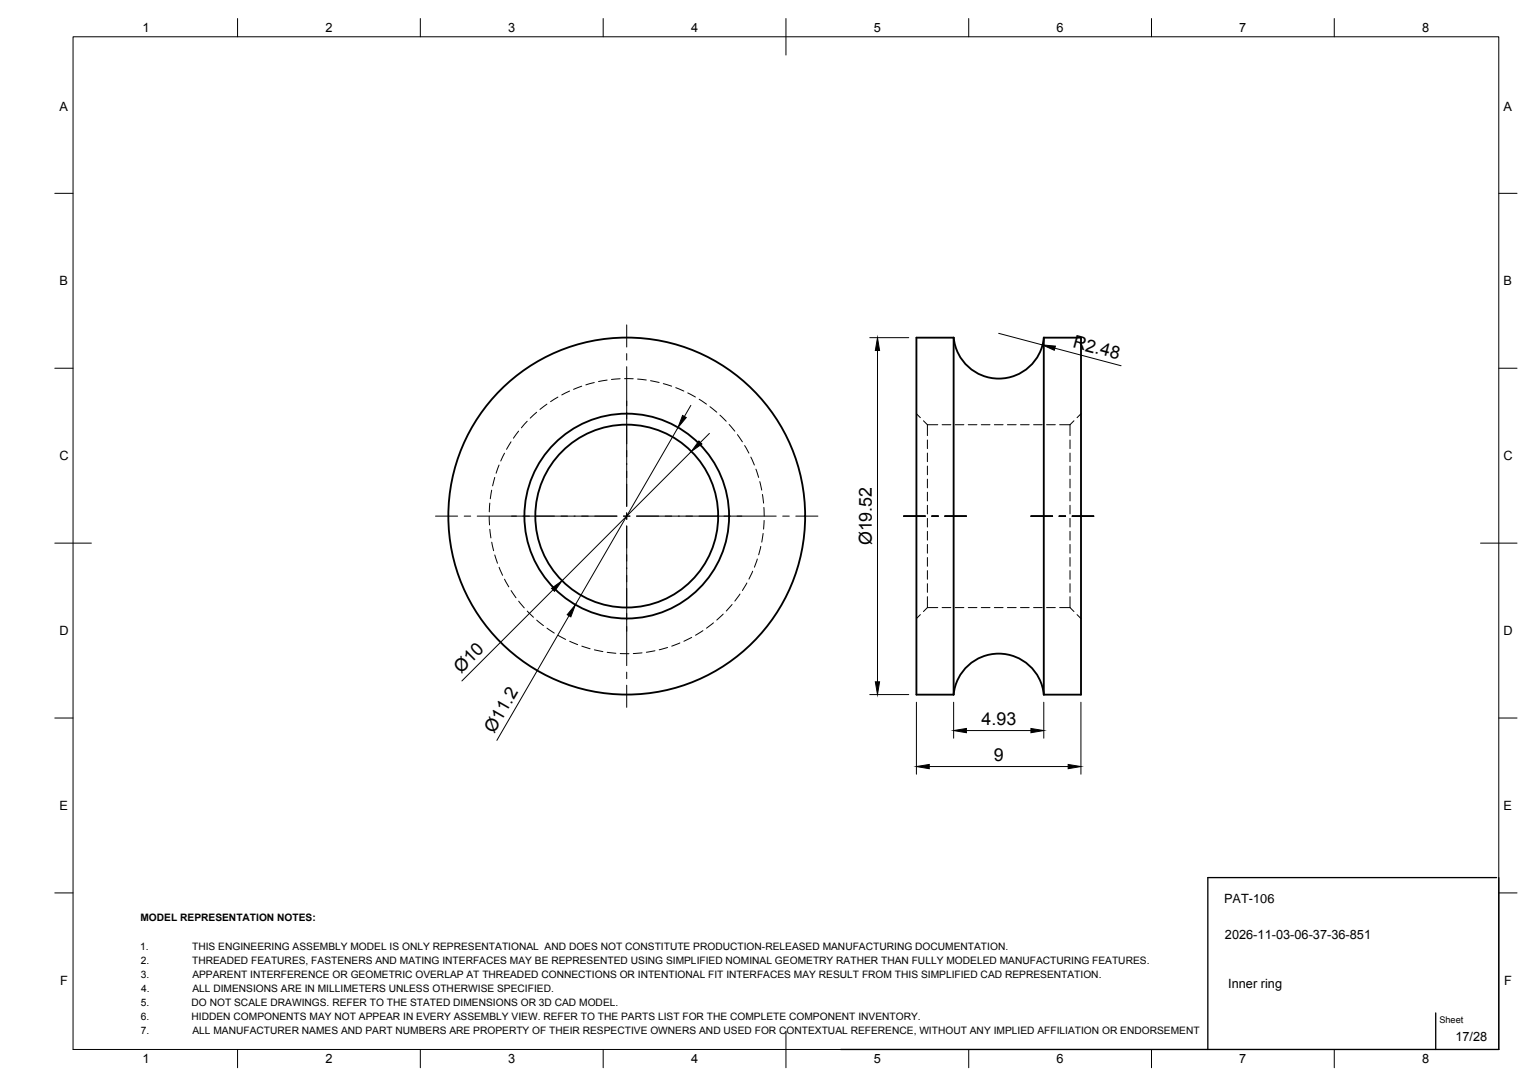
ISO-10303-21;
HEADER;
/* Generated by software containing ST-Developer
 * from STEP Tools, Inc. (www.steptools.com) 
 */

FILE_DESCRIPTION(
/* description */ ('Torsion-spring ratchet demonstrator'),
/* implementation_level */ '2;1');

FILE_NAME(
/* name */ 'Inner ring.step',
/* time_stamp */ '2026-10-29T17:29:17-07:00',
/* author */ (''),
/* organization */ (''),
/* preprocessor_version */ 'ST-DEVELOPER v20.2',
/* originating_system */ 'Autodesk Translation Framework v15.17.0.0',
/* authorisation */ '');

FILE_SCHEMA (('AUTOMOTIVE_DESIGN { 1 0 10303 214 3 1 1 }'));
ENDSEC;

DATA;
#10=MECHANICAL_DESIGN_GEOMETRIC_PRESENTATION_REPRESENTATION('',(#292),#11258);
#186=CONICAL_SURFACE('',#5693,0.53,0.785398163397448);
#187=CONICAL_SURFACE('',#5700,0.53,0.785398163397448);
#199=TOROIDAL_SURFACE('',#5682,1.,0.247676);
#244=SHAPE_REPRESENTATION_RELATIONSHIP('SRR','None',#11371,#268);
#268=ADVANCED_BREP_SHAPE_REPRESENTATION('',(#324),#11241);
#292=STYLED_ITEM('',(#11584),#324);
#324=MANIFOLD_SOLID_BREP('Body1',#5163);
#409=FACE_BOUND('',#1101,.T.);
#410=FACE_BOUND('',#1104,.T.);
#489=PLANE('',#5695);
#490=PLANE('',#5698);
#727=FACE_OUTER_BOUND('',#1096,.T.);
#728=FACE_OUTER_BOUND('',#1097,.T.);
#729=FACE_OUTER_BOUND('',#1098,.T.);
#730=FACE_OUTER_BOUND('',#1099,.T.);
#731=FACE_OUTER_BOUND('',#1100,.T.);
#732=FACE_OUTER_BOUND('',#1102,.T.);
#733=FACE_OUTER_BOUND('',#1103,.T.);
#734=FACE_OUTER_BOUND('',#1105,.T.);
#1096=EDGE_LOOP('',(#3862,#3863,#3864,#3865,#3866,#3867));
#1097=EDGE_LOOP('',(#3868,#3869,#3870,#3871,#3872));
#1098=EDGE_LOOP('',(#3873,#3874,#3875,#3876));
#1099=EDGE_LOOP('',(#3877,#3878,#3879,#3880));
#1100=EDGE_LOOP('',(#3881));
#1101=EDGE_LOOP('',(#3882));
#1102=EDGE_LOOP('',(#3883,#3884,#3885,#3886,#3887));
#1103=EDGE_LOOP('',(#3888));
#1104=EDGE_LOOP('',(#3889));
#1105=EDGE_LOOP('',(#3890,#3891,#3892,#3893));
#1419=LINE('',#8222,#1802);
#1420=LINE('',#8228,#1803);
#1421=LINE('',#8232,#1804);
#1422=LINE('',#8238,#1805);
#1423=LINE('',#8243,#1806);
#1802=VECTOR('',#6632,0.976185);
#1803=VECTOR('',#6639,0.5);
#1804=VECTOR('',#6644,0.53);
#1805=VECTOR('',#6653,0.976185);
#1806=VECTOR('',#6660,0.53);
#2203=CIRCLE('',#5683,0.976185);
#2204=CIRCLE('',#5684,0.976185);
#2205=CIRCLE('',#5685,0.247676);
#2206=CIRCLE('',#5686,0.976185);
#2207=CIRCLE('',#5687,0.976185);
#2208=CIRCLE('',#5689,0.976185);
#2209=CIRCLE('',#5691,0.5);
#2210=CIRCLE('',#5692,0.5);
#2211=CIRCLE('',#5694,0.56);
#2212=CIRCLE('',#5697,0.976185);
#2213=CIRCLE('',#5699,0.56);
#2475=VERTEX_POINT('',#8211);
#2476=VERTEX_POINT('',#8212);
#2477=VERTEX_POINT('',#8215);
#2478=VERTEX_POINT('',#8217);
#2479=VERTEX_POINT('',#8221);
#2480=VERTEX_POINT('',#8225);
#2481=VERTEX_POINT('',#8227);
#2482=VERTEX_POINT('',#8231);
#2483=VERTEX_POINT('',#8236);
#2484=VERTEX_POINT('',#8240);
#2991=EDGE_CURVE('',#2475,#2476,#2203,.T.);
#2992=EDGE_CURVE('',#2476,#2475,#2204,.T.);
#2993=EDGE_CURVE('',#2476,#2477,#2205,.T.);
#2994=EDGE_CURVE('',#2478,#2477,#2206,.T.);
#2995=EDGE_CURVE('',#2477,#2478,#2207,.T.);
#2996=EDGE_CURVE('',#2478,#2479,#1419,.T.);
#2997=EDGE_CURVE('',#2479,#2479,#2208,.T.);
#2998=EDGE_CURVE('',#2480,#2480,#2209,.T.);
#2999=EDGE_CURVE('',#2480,#2481,#1420,.T.);
#3000=EDGE_CURVE('',#2481,#2481,#2210,.T.);
#3001=EDGE_CURVE('',#2481,#2482,#1421,.T.);
#3002=EDGE_CURVE('',#2482,#2482,#2211,.T.);
#3003=EDGE_CURVE('',#2483,#2483,#2212,.T.);
#3004=EDGE_CURVE('',#2483,#2475,#1422,.T.);
#3005=EDGE_CURVE('',#2484,#2484,#2213,.T.);
#3006=EDGE_CURVE('',#2484,#2480,#1423,.T.);
#3862=ORIENTED_EDGE('',*,*,#2991,.F.);
#3863=ORIENTED_EDGE('',*,*,#2992,.F.);
#3864=ORIENTED_EDGE('',*,*,#2993,.T.);
#3865=ORIENTED_EDGE('',*,*,#2994,.F.);
#3866=ORIENTED_EDGE('',*,*,#2995,.F.);
#3867=ORIENTED_EDGE('',*,*,#2993,.F.);
#3868=ORIENTED_EDGE('',*,*,#2994,.T.);
#3869=ORIENTED_EDGE('',*,*,#2995,.T.);
#3870=ORIENTED_EDGE('',*,*,#2996,.T.);
#3871=ORIENTED_EDGE('',*,*,#2997,.T.);
#3872=ORIENTED_EDGE('',*,*,#2996,.F.);
#3873=ORIENTED_EDGE('',*,*,#2998,.T.);
#3874=ORIENTED_EDGE('',*,*,#2999,.T.);
#3875=ORIENTED_EDGE('',*,*,#3000,.F.);
#3876=ORIENTED_EDGE('',*,*,#2999,.F.);
#3877=ORIENTED_EDGE('',*,*,#3000,.T.);
#3878=ORIENTED_EDGE('',*,*,#3001,.T.);
#3879=ORIENTED_EDGE('',*,*,#3002,.F.);
#3880=ORIENTED_EDGE('',*,*,#3001,.F.);
#3881=ORIENTED_EDGE('',*,*,#2997,.F.);
#3882=ORIENTED_EDGE('',*,*,#3002,.T.);
#3883=ORIENTED_EDGE('',*,*,#3003,.F.);
#3884=ORIENTED_EDGE('',*,*,#3004,.T.);
#3885=ORIENTED_EDGE('',*,*,#2991,.T.);
#3886=ORIENTED_EDGE('',*,*,#2992,.T.);
#3887=ORIENTED_EDGE('',*,*,#3004,.F.);
#3888=ORIENTED_EDGE('',*,*,#3003,.T.);
#3889=ORIENTED_EDGE('',*,*,#3005,.F.);
#3890=ORIENTED_EDGE('',*,*,#3005,.T.);
#3891=ORIENTED_EDGE('',*,*,#3006,.T.);
#3892=ORIENTED_EDGE('',*,*,#2998,.F.);
#3893=ORIENTED_EDGE('',*,*,#3006,.F.);
#4816=CYLINDRICAL_SURFACE('',#5688,0.976185);
#4817=CYLINDRICAL_SURFACE('',#5690,0.5);
#4818=CYLINDRICAL_SURFACE('',#5696,0.976185);
#4953=ADVANCED_FACE('',(#727),#199,.F.);
#4954=ADVANCED_FACE('',(#728),#4816,.T.);
#4955=ADVANCED_FACE('',(#729),#4817,.F.);
#4956=ADVANCED_FACE('',(#730),#186,.F.);
#4957=ADVANCED_FACE('',(#731,#409),#489,.T.);
#4958=ADVANCED_FACE('',(#732),#4818,.T.);
#4959=ADVANCED_FACE('',(#733,#410),#490,.T.);
#4960=ADVANCED_FACE('',(#734),#187,.F.);
#5163=CLOSED_SHELL('',(#4953,#4954,#4955,#4956,#4957,#4958,#4959,#4960));
#5681=AXIS2_PLACEMENT_3D('',#8209,#6616,#6617);
#5682=AXIS2_PLACEMENT_3D('',#8210,#6618,#6619);
#5683=AXIS2_PLACEMENT_3D('',#8213,#6620,#6621);
#5684=AXIS2_PLACEMENT_3D('',#8214,#6622,#6623);
#5685=AXIS2_PLACEMENT_3D('',#8216,#6624,#6625);
#5686=AXIS2_PLACEMENT_3D('',#8218,#6626,#6627);
#5687=AXIS2_PLACEMENT_3D('',#8219,#6628,#6629);
#5688=AXIS2_PLACEMENT_3D('',#8220,#6630,#6631);
#5689=AXIS2_PLACEMENT_3D('',#8223,#6633,#6634);
#5690=AXIS2_PLACEMENT_3D('',#8224,#6635,#6636);
#5691=AXIS2_PLACEMENT_3D('',#8226,#6637,#6638);
#5692=AXIS2_PLACEMENT_3D('',#8229,#6640,#6641);
#5693=AXIS2_PLACEMENT_3D('',#8230,#6642,#6643);
#5694=AXIS2_PLACEMENT_3D('',#8233,#6645,#6646);
#5695=AXIS2_PLACEMENT_3D('',#8234,#6647,#6648);
#5696=AXIS2_PLACEMENT_3D('',#8235,#6649,#6650);
#5697=AXIS2_PLACEMENT_3D('',#8237,#6651,#6652);
#5698=AXIS2_PLACEMENT_3D('',#8239,#6654,#6655);
#5699=AXIS2_PLACEMENT_3D('',#8241,#6656,#6657);
#5700=AXIS2_PLACEMENT_3D('',#8242,#6658,#6659);
#6616=DIRECTION('axis',(0.,0.,1.));
#6617=DIRECTION('refdir',(1.,0.,0.));
#6618=DIRECTION('center_axis',(0.,-1.,0.));
#6619=DIRECTION('ref_axis',(0.,0.,-1.));
#6620=DIRECTION('center_axis',(0.,-1.,0.));
#6621=DIRECTION('ref_axis',(1.,0.,0.));
#6622=DIRECTION('center_axis',(0.,-1.,0.));
#6623=DIRECTION('ref_axis',(1.,0.,0.));
#6624=DIRECTION('center_axis',(1.,0.,1.22464679914735E-16));
#6625=DIRECTION('ref_axis',(-1.22464679914735E-16,0.,1.));
#6626=DIRECTION('center_axis',(0.,1.,0.));
#6627=DIRECTION('ref_axis',(1.,0.,0.));
#6628=DIRECTION('center_axis',(0.,1.,0.));
#6629=DIRECTION('ref_axis',(1.,0.,0.));
#6630=DIRECTION('center_axis',(0.,-1.,0.));
#6631=DIRECTION('ref_axis',(1.,0.,0.));
#6632=DIRECTION('',(0.,1.,0.));
#6633=DIRECTION('center_axis',(0.,-1.,0.));
#6634=DIRECTION('ref_axis',(1.,0.,0.));
#6635=DIRECTION('center_axis',(0.,-1.,0.));
#6636=DIRECTION('ref_axis',(1.,0.,0.));
#6637=DIRECTION('center_axis',(0.,-1.,0.));
#6638=DIRECTION('ref_axis',(1.,0.,0.));
#6639=DIRECTION('',(0.,1.,0.));
#6640=DIRECTION('center_axis',(0.,-1.,0.));
#6641=DIRECTION('ref_axis',(1.,0.,0.));
#6642=DIRECTION('center_axis',(0.,1.,0.));
#6643=DIRECTION('ref_axis',(1.,0.,0.));
#6644=DIRECTION('',(-0.707106781186547,0.707106781186548,-8.65956056235493E-17));
#6645=DIRECTION('center_axis',(0.,-1.,0.));
#6646=DIRECTION('ref_axis',(1.,0.,0.));
#6647=DIRECTION('center_axis',(0.,1.,0.));
#6648=DIRECTION('ref_axis',(0.,0.,1.));
#6649=DIRECTION('center_axis',(0.,-1.,0.));
#6650=DIRECTION('ref_axis',(1.,0.,0.));
#6651=DIRECTION('center_axis',(0.,-1.,0.));
#6652=DIRECTION('ref_axis',(1.,0.,0.));
#6653=DIRECTION('',(0.,1.,0.));
#6654=DIRECTION('center_axis',(0.,-1.,0.));
#6655=DIRECTION('ref_axis',(0.,0.,-1.));
#6656=DIRECTION('center_axis',(0.,-1.,0.));
#6657=DIRECTION('ref_axis',(1.,0.,0.));
#6658=DIRECTION('center_axis',(0.,-1.,0.));
#6659=DIRECTION('ref_axis',(1.,0.,0.));
#6660=DIRECTION('',(0.707106781186547,0.707106781186548,8.65956056235493E-17));
#8209=CARTESIAN_POINT('',(0.,0.,0.));
#8210=CARTESIAN_POINT('Origin',(0.,0.,0.));
#8211=CARTESIAN_POINT('',(-0.976185,-0.246528389340863,-1.19548183562566E-16));
#8212=CARTESIAN_POINT('',(-1.19548183562566E-16,-0.246528389340863,0.976185));
#8213=CARTESIAN_POINT('Origin',(0.,-0.246528389340863,0.));
#8214=CARTESIAN_POINT('Origin',(0.,-0.246528389340863,0.));
#8215=CARTESIAN_POINT('',(-1.19548183562566E-16,0.246528389340863,0.976185));
#8216=CARTESIAN_POINT('Origin',(-1.22464679914735E-16,0.,1.));
#8217=CARTESIAN_POINT('',(-0.976185,0.246528389340863,1.19548183562566E-16));
#8218=CARTESIAN_POINT('Origin',(0.,0.246528389340863,0.));
#8219=CARTESIAN_POINT('Origin',(0.,0.246528389340863,0.));
#8220=CARTESIAN_POINT('Origin',(0.,0.,0.));
#8221=CARTESIAN_POINT('',(-0.976185,0.45,-1.19548183562566E-16));
#8222=CARTESIAN_POINT('',(-0.976185,0.,-1.19548183562566E-16));
#8223=CARTESIAN_POINT('Origin',(0.,0.45,0.));
#8224=CARTESIAN_POINT('Origin',(0.,0.,0.));
#8225=CARTESIAN_POINT('',(-0.5,-0.39,-6.12323399573677E-17));
#8226=CARTESIAN_POINT('Origin',(0.,-0.39,0.));
#8227=CARTESIAN_POINT('',(-0.5,0.39,-6.12323399573677E-17));
#8228=CARTESIAN_POINT('',(-0.5,0.,-6.12323399573677E-17));
#8229=CARTESIAN_POINT('Origin',(0.,0.39,0.));
#8230=CARTESIAN_POINT('Origin',(0.,0.42,0.));
#8231=CARTESIAN_POINT('',(-0.56,0.45,-6.85802207522518E-17));
#8232=CARTESIAN_POINT('',(-0.53,0.42,-6.49062803548097E-17));
#8233=CARTESIAN_POINT('Origin',(0.,0.45,0.));
#8234=CARTESIAN_POINT('Origin',(0.976185,0.45,0.));
#8235=CARTESIAN_POINT('Origin',(0.,0.,0.));
#8236=CARTESIAN_POINT('',(-0.976185,-0.45,-1.19548183562566E-16));
#8237=CARTESIAN_POINT('Origin',(0.,-0.45,0.));
#8238=CARTESIAN_POINT('',(-0.976185,0.,-1.19548183562566E-16));
#8239=CARTESIAN_POINT('Origin',(0.56,-0.45,0.));
#8240=CARTESIAN_POINT('',(-0.56,-0.45,-6.85802207522518E-17));
#8241=CARTESIAN_POINT('Origin',(0.,-0.45,0.));
#8242=CARTESIAN_POINT('Origin',(0.,-0.42,0.));
#8243=CARTESIAN_POINT('',(-0.53,-0.42,-6.49062803548097E-17));
#11211=UNCERTAINTY_MEASURE_WITH_UNIT(LENGTH_MEASURE(0.001),#11259,
'DISTANCE_ACCURACY_VALUE',
'Maximum model space distance between geometric entities at asserted c
onnectivities');
#11228=UNCERTAINTY_MEASURE_WITH_UNIT(LENGTH_MEASURE(0.001),#11259,
'DISTANCE_ACCURACY_VALUE',
'Maximum model space distance between geometric entities at asserted c
onnectivities');
#11241=(
GEOMETRIC_REPRESENTATION_CONTEXT(3)
GLOBAL_UNCERTAINTY_ASSIGNED_CONTEXT((#11211))
GLOBAL_UNIT_ASSIGNED_CONTEXT((#11259,#11261,#11262))
REPRESENTATION_CONTEXT('','3D')
);
#11258=(
GEOMETRIC_REPRESENTATION_CONTEXT(3)
GLOBAL_UNCERTAINTY_ASSIGNED_CONTEXT((#11228))
GLOBAL_UNIT_ASSIGNED_CONTEXT((#11259,#11261,#11262))
REPRESENTATION_CONTEXT('','3D')
);
#11259=(
LENGTH_UNIT()
NAMED_UNIT(*)
SI_UNIT(.CENTI.,.METRE.)
);
#11261=(
NAMED_UNIT(*)
PLANE_ANGLE_UNIT()
SI_UNIT($,.RADIAN.)
);
#11262=(
NAMED_UNIT(*)
SI_UNIT($,.STERADIAN.)
SOLID_ANGLE_UNIT()
);
#11275=SHAPE_DEFINITION_REPRESENTATION(#11304,#11371);
#11304=PRODUCT_DEFINITION_SHAPE('',$,#11401);
#11371=SHAPE_REPRESENTATION('',(#5681),#11241);
#11388=PRODUCT_DEFINITION_CONTEXT('part definition',#11477,'design');
#11401=PRODUCT_DEFINITION('Inner ring','Inner ring',#11430,#11388);
#11430=PRODUCT_DEFINITION_FORMATION('',$,#11491);
#11477=APPLICATION_CONTEXT(
'Core Data for Automotive Mechanical Design Process');
#11478=PRODUCT_CONTEXT('part definition',#11477,'mechanical');
#11491=PRODUCT('Inner ring','Inner ring','Inner ring',(#11478));
#11578=COLOUR_RGB('Grey',0.48,0.52,0.57);
#11579=FILL_AREA_STYLE_COLOUR('',#11578);
#11580=FILL_AREA_STYLE('',(#11579));
#11581=SURFACE_STYLE_FILL_AREA(#11580);
#11582=SURFACE_SIDE_STYLE('',(#11581));
#11583=SURFACE_STYLE_USAGE(.BOTH.,#11582);
#11584=PRESENTATION_STYLE_ASSIGNMENT((#11583));
ENDSEC;
END-ISO-10303-21;
